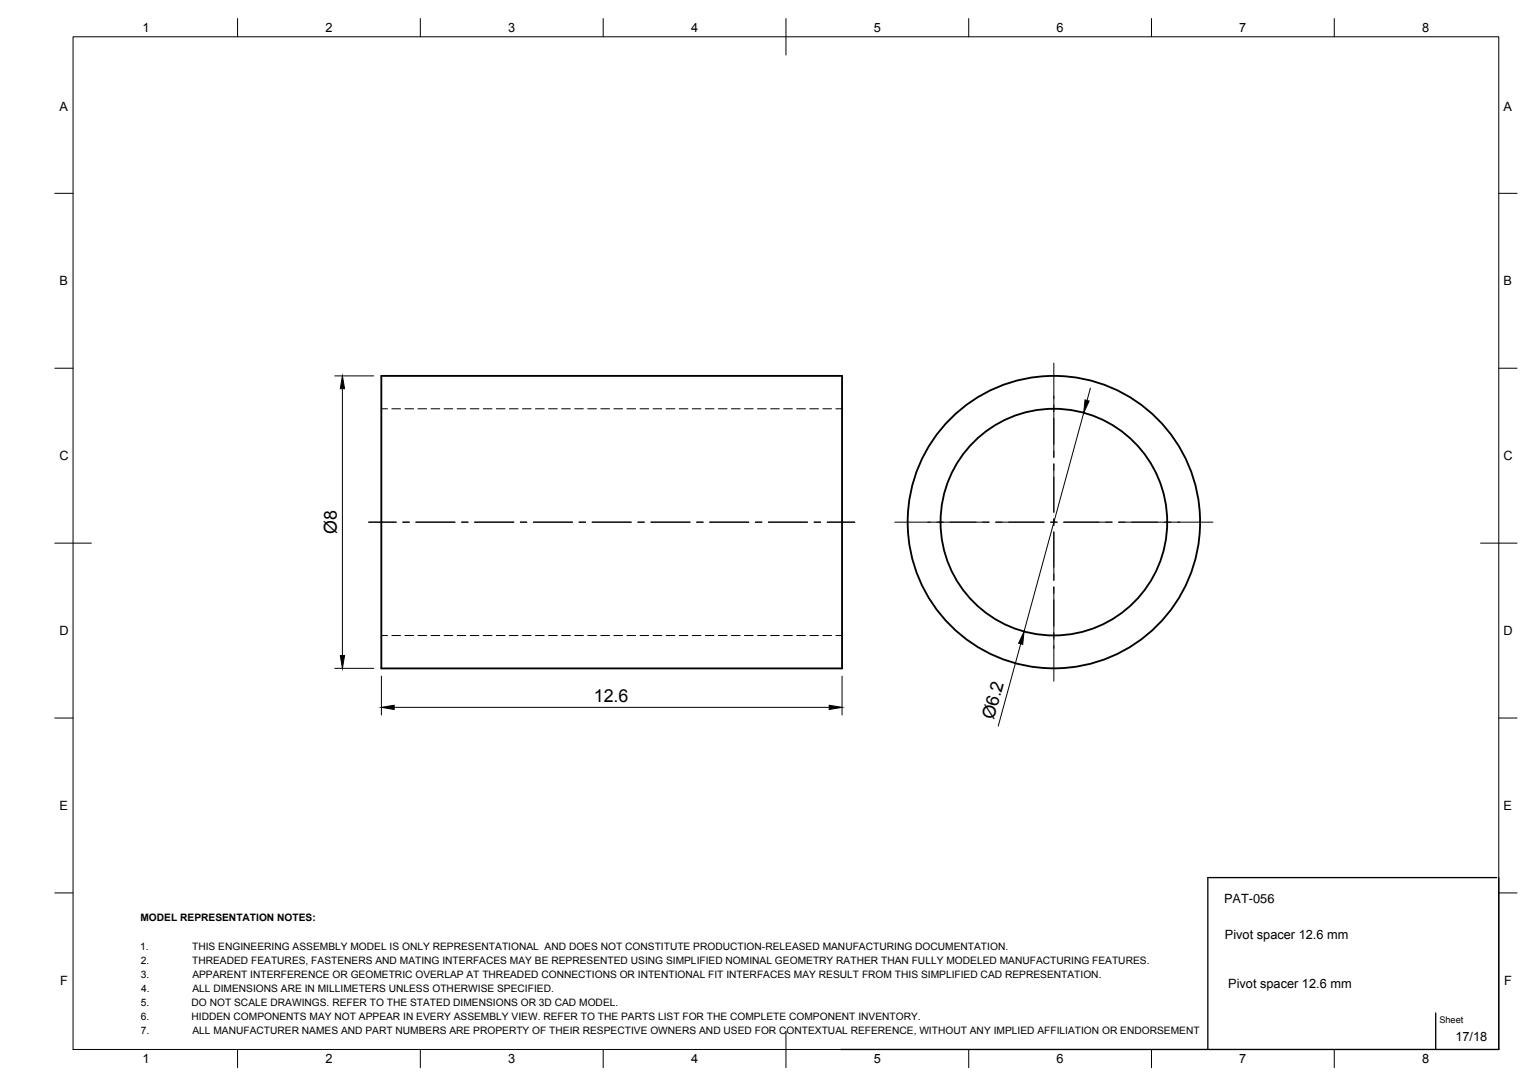
ISO-10303-21;
HEADER;
/* Generated by software containing ST-Developer
 * from STEP Tools, Inc. (www.steptools.com) 
 */

FILE_DESCRIPTION(
/* description */ ('Hook toggle clamp'),
/* implementation_level */ '2;1');

FILE_NAME(
/* name */ 'Pivot spacer 12.6 mm.step',
/* time_stamp */ '2026-10-27T21:56:56-07:00',
/* author */ (''),
/* organization */ (''),
/* preprocessor_version */ 'ST-DEVELOPER v20.2',
/* originating_system */ 'Autodesk Translation Framework v15.17.0.0',
/* authorisation */ '');

FILE_SCHEMA (('AUTOMOTIVE_DESIGN { 1 0 10303 214 3 1 1 }'));
ENDSEC;

DATA;
#10=MECHANICAL_DESIGN_GEOMETRIC_PRESENTATION_REPRESENTATION('',(#199),#5458);
#165=SHAPE_REPRESENTATION_RELATIONSHIP('SRR','None',#5549,#182);
#182=ADVANCED_BREP_SHAPE_REPRESENTATION('',(#215),#5451);
#199=STYLED_ITEM('',(#5710),#215);
#215=MANIFOLD_SOLID_BREP('Body1',#2981);
#267=FACE_BOUND('',#746,.T.);
#268=FACE_BOUND('',#748,.T.);
#371=PLANE('',#3410);
#372=PLANE('',#3411);
#525=FACE_OUTER_BOUND('',#743,.T.);
#526=FACE_OUTER_BOUND('',#744,.T.);
#527=FACE_OUTER_BOUND('',#745,.T.);
#528=FACE_OUTER_BOUND('',#747,.T.);
#743=EDGE_LOOP('',(#2589,#2590,#2591,#2592));
#744=EDGE_LOOP('',(#2593,#2594,#2595,#2596));
#745=EDGE_LOOP('',(#2597));
#746=EDGE_LOOP('',(#2598));
#747=EDGE_LOOP('',(#2599));
#748=EDGE_LOOP('',(#2600));
#1004=LINE('',#5070,#1241);
#1005=LINE('',#5076,#1242);
#1241=VECTOR('',#4180,0.31);
#1242=VECTOR('',#4187,0.4);
#1348=CIRCLE('',#3405,0.31);
#1349=CIRCLE('',#3406,0.31);
#1350=CIRCLE('',#3408,0.4);
#1351=CIRCLE('',#3409,0.4);
#1575=VERTEX_POINT('',#5067);
#1576=VERTEX_POINT('',#5069);
#1577=VERTEX_POINT('',#5073);
#1578=VERTEX_POINT('',#5075);
#1921=EDGE_CURVE('',#1575,#1575,#1348,.T.);
#1922=EDGE_CURVE('',#1575,#1576,#1004,.T.);
#1923=EDGE_CURVE('',#1576,#1576,#1349,.T.);
#1924=EDGE_CURVE('',#1577,#1577,#1350,.T.);
#1925=EDGE_CURVE('',#1577,#1578,#1005,.T.);
#1926=EDGE_CURVE('',#1578,#1578,#1351,.T.);
#2589=ORIENTED_EDGE('',*,*,#1921,.F.);
#2590=ORIENTED_EDGE('',*,*,#1922,.T.);
#2591=ORIENTED_EDGE('',*,*,#1923,.T.);
#2592=ORIENTED_EDGE('',*,*,#1922,.F.);
#2593=ORIENTED_EDGE('',*,*,#1924,.F.);
#2594=ORIENTED_EDGE('',*,*,#1925,.T.);
#2595=ORIENTED_EDGE('',*,*,#1926,.T.);
#2596=ORIENTED_EDGE('',*,*,#1925,.F.);
#2597=ORIENTED_EDGE('',*,*,#1924,.T.);
#2598=ORIENTED_EDGE('',*,*,#1921,.T.);
#2599=ORIENTED_EDGE('',*,*,#1926,.F.);
#2600=ORIENTED_EDGE('',*,*,#1923,.F.);
#2784=CYLINDRICAL_SURFACE('',#3404,0.31);
#2785=CYLINDRICAL_SURFACE('',#3407,0.4);
#2929=ADVANCED_FACE('',(#525),#2784,.F.);
#2930=ADVANCED_FACE('',(#526),#2785,.T.);
#2931=ADVANCED_FACE('',(#527,#267),#371,.T.);
#2932=ADVANCED_FACE('',(#528,#268),#372,.F.);
#2981=CLOSED_SHELL('',(#2929,#2930,#2931,#2932));
#3403=AXIS2_PLACEMENT_3D('',#5065,#4174,#4175);
#3404=AXIS2_PLACEMENT_3D('',#5066,#4176,#4177);
#3405=AXIS2_PLACEMENT_3D('',#5068,#4178,#4179);
#3406=AXIS2_PLACEMENT_3D('',#5071,#4181,#4182);
#3407=AXIS2_PLACEMENT_3D('',#5072,#4183,#4184);
#3408=AXIS2_PLACEMENT_3D('',#5074,#4185,#4186);
#3409=AXIS2_PLACEMENT_3D('',#5077,#4188,#4189);
#3410=AXIS2_PLACEMENT_3D('',#5078,#4190,#4191);
#3411=AXIS2_PLACEMENT_3D('',#5079,#4192,#4193);
#4174=DIRECTION('axis',(0.,0.,1.));
#4175=DIRECTION('refdir',(1.,0.,0.));
#4176=DIRECTION('center_axis',(0.,1.,0.));
#4177=DIRECTION('ref_axis',(1.,0.,0.));
#4178=DIRECTION('center_axis',(0.,-1.,0.));
#4179=DIRECTION('ref_axis',(1.,0.,0.));
#4180=DIRECTION('',(0.,-1.,0.));
#4181=DIRECTION('center_axis',(0.,-1.,0.));
#4182=DIRECTION('ref_axis',(1.,0.,0.));
#4183=DIRECTION('center_axis',(0.,1.,0.));
#4184=DIRECTION('ref_axis',(1.,0.,0.));
#4185=DIRECTION('center_axis',(0.,1.,0.));
#4186=DIRECTION('ref_axis',(1.,0.,0.));
#4187=DIRECTION('',(0.,-1.,0.));
#4188=DIRECTION('center_axis',(0.,1.,0.));
#4189=DIRECTION('ref_axis',(1.,0.,0.));
#4190=DIRECTION('center_axis',(0.,1.,0.));
#4191=DIRECTION('ref_axis',(1.,0.,0.));
#4192=DIRECTION('center_axis',(0.,1.,0.));
#4193=DIRECTION('ref_axis',(1.,0.,0.));
#5065=CARTESIAN_POINT('',(0.,0.,0.));
#5066=CARTESIAN_POINT('Origin',(2.00423507354465,-0.32,2.5));
#5067=CARTESIAN_POINT('',(1.69423507354465,0.94,2.5));
#5068=CARTESIAN_POINT('Origin',(2.00423507354465,0.94,2.5));
#5069=CARTESIAN_POINT('',(1.69423507354465,-0.32,2.5));
#5070=CARTESIAN_POINT('',(1.69423507354465,-0.32,2.5));
#5071=CARTESIAN_POINT('Origin',(2.00423507354465,-0.32,2.5));
#5072=CARTESIAN_POINT('Origin',(2.00423507354465,-0.32,2.5));
#5073=CARTESIAN_POINT('',(1.60423507354465,0.94,2.5));
#5074=CARTESIAN_POINT('Origin',(2.00423507354465,0.94,2.5));
#5075=CARTESIAN_POINT('',(1.60423507354465,-0.32,2.5));
#5076=CARTESIAN_POINT('',(1.60423507354465,-0.32,2.5));
#5077=CARTESIAN_POINT('Origin',(2.00423507354465,-0.32,2.5));
#5078=CARTESIAN_POINT('Origin',(2.00423507354465,0.94,2.5));
#5079=CARTESIAN_POINT('Origin',(2.00423507354465,-0.32,2.5));
#5428=UNCERTAINTY_MEASURE_WITH_UNIT(LENGTH_MEASURE(0.001),#5459,
'DISTANCE_ACCURACY_VALUE',
'Maximum model space distance between geometric entities at asserted c
onnectivities');
#5435=UNCERTAINTY_MEASURE_WITH_UNIT(LENGTH_MEASURE(0.001),#5459,
'DISTANCE_ACCURACY_VALUE',
'Maximum model space distance between geometric entities at asserted c
onnectivities');
#5451=(
GEOMETRIC_REPRESENTATION_CONTEXT(3)
GLOBAL_UNCERTAINTY_ASSIGNED_CONTEXT((#5428))
GLOBAL_UNIT_ASSIGNED_CONTEXT((#5459,#5461,#5462))
REPRESENTATION_CONTEXT('','3D')
);
#5458=(
GEOMETRIC_REPRESENTATION_CONTEXT(3)
GLOBAL_UNCERTAINTY_ASSIGNED_CONTEXT((#5435))
GLOBAL_UNIT_ASSIGNED_CONTEXT((#5459,#5461,#5462))
REPRESENTATION_CONTEXT('','3D')
);
#5459=(
LENGTH_UNIT()
NAMED_UNIT(*)
SI_UNIT(.CENTI.,.METRE.)
);
#5461=(
NAMED_UNIT(*)
PLANE_ANGLE_UNIT()
SI_UNIT($,.RADIAN.)
);
#5462=(
NAMED_UNIT(*)
SI_UNIT($,.STERADIAN.)
SOLID_ANGLE_UNIT()
);
#5478=SHAPE_DEFINITION_REPRESENTATION(#5501,#5549);
#5501=PRODUCT_DEFINITION_SHAPE('',$,#5572);
#5549=SHAPE_REPRESENTATION('',(#3403),#5451);
#5556=PRODUCT_DEFINITION_CONTEXT('part definition',#5624,'design');
#5572=PRODUCT_DEFINITION('Pivot spacer 12.6 mm','Pivot spacer 12.6 mm',
#5594,#5556);
#5594=PRODUCT_DEFINITION_FORMATION('',$,#5641);
#5624=APPLICATION_CONTEXT(
'Core Data for Automotive Mechanical Design Process');
#5625=PRODUCT_CONTEXT('part definition',#5624,'mechanical');
#5641=PRODUCT('Pivot spacer 12.6 mm','Pivot spacer 12.6 mm',
'Pivot spacer 12.6 mm',(#5625));
#5704=COLOUR_RGB('Sky Blue',0.24,0.69,0.87);
#5705=FILL_AREA_STYLE_COLOUR('',#5704);
#5706=FILL_AREA_STYLE('',(#5705));
#5707=SURFACE_STYLE_FILL_AREA(#5706);
#5708=SURFACE_SIDE_STYLE('',(#5707));
#5709=SURFACE_STYLE_USAGE(.BOTH.,#5708);
#5710=PRESENTATION_STYLE_ASSIGNMENT((#5709));
ENDSEC;
END-ISO-10303-21;
